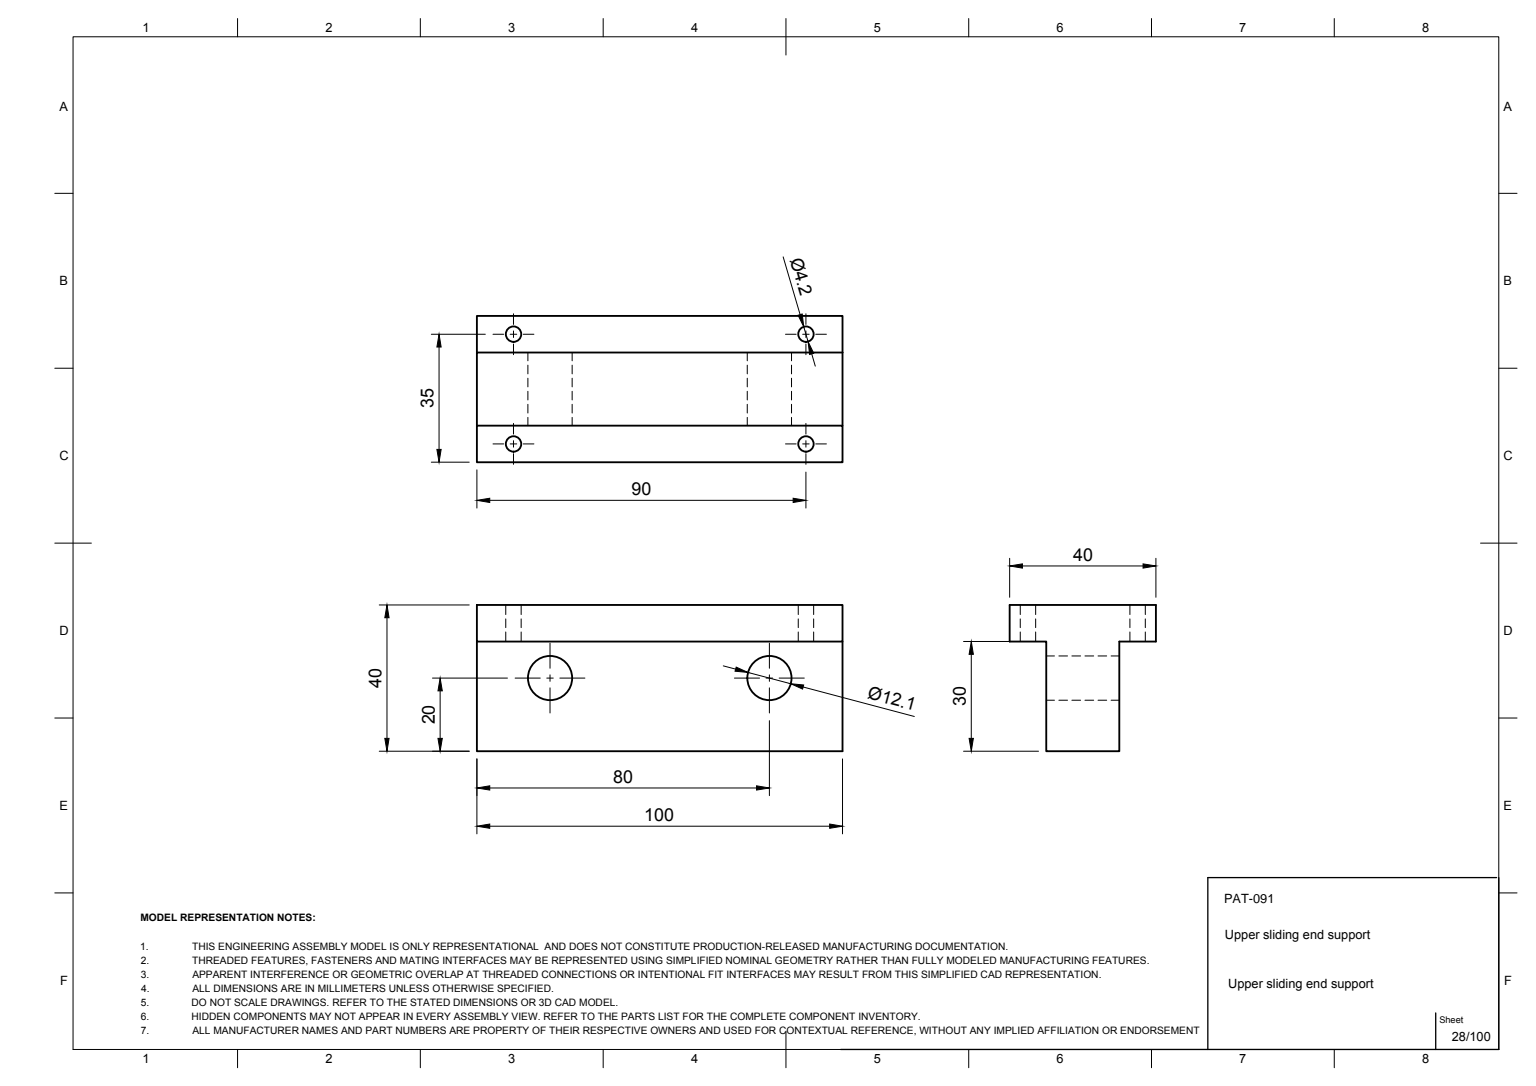
ISO-10303-21;
HEADER;
/* Generated by software containing ST-Developer
 * from STEP Tools, Inc. (www.steptools.com) 
 */

FILE_DESCRIPTION(
/* description */ ('PAT-091'),
/* implementation_level */ '2;1');

FILE_NAME(
/* name */ 'Upper sliding end support.step',
/* time_stamp */ '2026-10-27T15:34:44-07:00',
/* author */ (''),
/* organization */ (''),
/* preprocessor_version */ 'ST-DEVELOPER v20.2',
/* originating_system */ 'Autodesk Translation Framework v15.17.0.0',
/* authorisation */ '');

FILE_SCHEMA (('AUTOMOTIVE_DESIGN { 1 0 10303 214 3 1 1 }'));
ENDSEC;

DATA;
#10=MECHANICAL_DESIGN_GEOMETRIC_PRESENTATION_REPRESENTATION('',(#991),#25100);
#771=SHAPE_REPRESENTATION_RELATIONSHIP('SRR','None',#25533,#881);
#881=ADVANCED_BREP_SHAPE_REPRESENTATION('',(#1114),#25003);
#991=STYLED_ITEM('',(#26184),#1114);
#1114=MANIFOLD_SOLID_BREP('Body1',#13269);
#1365=FACE_BOUND('',#3226,.T.);
#1366=FACE_BOUND('',#3227,.T.);
#1367=FACE_BOUND('',#3231,.T.);
#1368=FACE_BOUND('',#3232,.T.);
#1369=FACE_BOUND('',#3234,.T.);
#1370=FACE_BOUND('',#3235,.T.);
#1371=FACE_BOUND('',#3241,.T.);
#1372=FACE_BOUND('',#3242,.T.);
#1373=FACE_BOUND('',#3244,.T.);
#1374=FACE_BOUND('',#3245,.T.);
#1375=FACE_BOUND('',#3246,.T.);
#1376=FACE_BOUND('',#3247,.T.);
#1736=PLANE('',#14996);
#1737=PLANE('',#14997);
#1738=PLANE('',#14998);
#1739=PLANE('',#14999);
#1740=PLANE('',#15000);
#1741=PLANE('',#15003);
#1742=PLANE('',#15008);
#1743=PLANE('',#15009);
#1744=PLANE('',#15010);
#1745=PLANE('',#15011);
#2253=FACE_OUTER_BOUND('',#3221,.T.);
#2254=FACE_OUTER_BOUND('',#3222,.T.);
#2255=FACE_OUTER_BOUND('',#3223,.T.);
#2256=FACE_OUTER_BOUND('',#3224,.T.);
#2257=FACE_OUTER_BOUND('',#3225,.T.);
#2258=FACE_OUTER_BOUND('',#3228,.T.);
#2259=FACE_OUTER_BOUND('',#3229,.T.);
#2260=FACE_OUTER_BOUND('',#3230,.T.);
#2261=FACE_OUTER_BOUND('',#3233,.T.);
#2262=FACE_OUTER_BOUND('',#3236,.T.);
#2263=FACE_OUTER_BOUND('',#3237,.T.);
#2264=FACE_OUTER_BOUND('',#3238,.T.);
#2265=FACE_OUTER_BOUND('',#3239,.T.);
#2266=FACE_OUTER_BOUND('',#3240,.T.);
#2267=FACE_OUTER_BOUND('',#3243,.T.);
#2268=FACE_OUTER_BOUND('',#3248,.T.);
#3221=EDGE_LOOP('',(#9806,#9807,#9808,#9809));
#3222=EDGE_LOOP('',(#9810,#9811,#9812,#9813));
#3223=EDGE_LOOP('',(#9814,#9815,#9816,#9817));
#3224=EDGE_LOOP('',(#9818,#9819,#9820,#9821));
#3225=EDGE_LOOP('',(#9822,#9823,#9824,#9825));
#3226=EDGE_LOOP('',(#9826));
#3227=EDGE_LOOP('',(#9827));
#3228=EDGE_LOOP('',(#9828,#9829,#9830,#9831));
#3229=EDGE_LOOP('',(#9832,#9833,#9834,#9835));
#3230=EDGE_LOOP('',(#9836,#9837,#9838,#9839));
#3231=EDGE_LOOP('',(#9840));
#3232=EDGE_LOOP('',(#9841));
#3233=EDGE_LOOP('',(#9842,#9843,#9844,#9845));
#3234=EDGE_LOOP('',(#9846));
#3235=EDGE_LOOP('',(#9847));
#3236=EDGE_LOOP('',(#9848,#9849,#9850,#9851,#9852,#9853,#9854,#9855));
#3237=EDGE_LOOP('',(#9856,#9857,#9858,#9859));
#3238=EDGE_LOOP('',(#9860,#9861,#9862,#9863));
#3239=EDGE_LOOP('',(#9864,#9865,#9866,#9867,#9868,#9869,#9870,#9871));
#3240=EDGE_LOOP('',(#9872,#9873,#9874,#9875));
#3241=EDGE_LOOP('',(#9876));
#3242=EDGE_LOOP('',(#9877));
#3243=EDGE_LOOP('',(#9878,#9879,#9880,#9881));
#3244=EDGE_LOOP('',(#9882));
#3245=EDGE_LOOP('',(#9883));
#3246=EDGE_LOOP('',(#9884));
#3247=EDGE_LOOP('',(#9885));
#3248=EDGE_LOOP('',(#9886,#9887,#9888,#9889));
#4356=LINE('',#21886,#5096);
#4357=LINE('',#21892,#5097);
#4358=LINE('',#21898,#5098);
#4359=LINE('',#21904,#5099);
#4360=LINE('',#21909,#5100);
#4361=LINE('',#21911,#5101);
#4362=LINE('',#21913,#5102);
#4363=LINE('',#21914,#5103);
#4364=LINE('',#21918,#5104);
#4365=LINE('',#21920,#5105);
#4366=LINE('',#21922,#5106);
#4367=LINE('',#21923,#5107);
#4368=LINE('',#21926,#5108);
#4369=LINE('',#21928,#5109);
#4370=LINE('',#21929,#5110);
#4371=LINE('',#21933,#5111);
#4372=LINE('',#21934,#5112);
#4373=LINE('',#21935,#5113);
#4374=LINE('',#21938,#5114);
#4375=LINE('',#21940,#5115);
#4376=LINE('',#21941,#5116);
#4377=LINE('',#21948,#5117);
#4378=LINE('',#21949,#5118);
#4379=LINE('',#21950,#5119);
#4380=LINE('',#21954,#5120);
#4381=LINE('',#21958,#5121);
#4382=LINE('',#21961,#5122);
#4383=LINE('',#21962,#5123);
#4384=LINE('',#21963,#5124);
#4385=LINE('',#21965,#5125);
#5096=VECTOR('',#17502,0.210000000000001);
#5097=VECTOR('',#17509,0.210000000000001);
#5098=VECTOR('',#17516,0.210000000000001);
#5099=VECTOR('',#17523,0.210000000000001);
#5100=VECTOR('',#17528,1.);
#5101=VECTOR('',#17529,1.);
#5102=VECTOR('',#17530,1.);
#5103=VECTOR('',#17531,1.);
#5104=VECTOR('',#17534,1.);
#5105=VECTOR('',#17535,1.);
#5106=VECTOR('',#17536,1.);
#5107=VECTOR('',#17537,1.);
#5108=VECTOR('',#17540,1.);
#5109=VECTOR('',#17541,1.);
#5110=VECTOR('',#17542,1.);
#5111=VECTOR('',#17545,1.);
#5112=VECTOR('',#17546,1.);
#5113=VECTOR('',#17547,1.);
#5114=VECTOR('',#17550,1.);
#5115=VECTOR('',#17551,1.);
#5116=VECTOR('',#17552,1.);
#5117=VECTOR('',#17559,1.);
#5118=VECTOR('',#17560,1.);
#5119=VECTOR('',#17561,1.);
#5120=VECTOR('',#17566,0.605);
#5121=VECTOR('',#17571,0.605);
#5122=VECTOR('',#17574,1.);
#5123=VECTOR('',#17575,1.);
#5124=VECTOR('',#17576,1.);
#5125=VECTOR('',#17579,1.);
#5789=CIRCLE('',#14985,0.210000000000001);
#5790=CIRCLE('',#14986,0.210000000000001);
#5791=CIRCLE('',#14988,0.210000000000001);
#5792=CIRCLE('',#14989,0.210000000000001);
#5793=CIRCLE('',#14991,0.210000000000001);
#5794=CIRCLE('',#14992,0.210000000000001);
#5795=CIRCLE('',#14994,0.210000000000001);
#5796=CIRCLE('',#14995,0.210000000000001);
#5797=CIRCLE('',#15001,0.605);
#5798=CIRCLE('',#15002,0.605);
#5799=CIRCLE('',#15005,0.605);
#5800=CIRCLE('',#15007,0.605);
#6660=VERTEX_POINT('',#21883);
#6661=VERTEX_POINT('',#21885);
#6662=VERTEX_POINT('',#21889);
#6663=VERTEX_POINT('',#21891);
#6664=VERTEX_POINT('',#21895);
#6665=VERTEX_POINT('',#21897);
#6666=VERTEX_POINT('',#21901);
#6667=VERTEX_POINT('',#21903);
#6668=VERTEX_POINT('',#21907);
#6669=VERTEX_POINT('',#21908);
#6670=VERTEX_POINT('',#21910);
#6671=VERTEX_POINT('',#21912);
#6672=VERTEX_POINT('',#21916);
#6673=VERTEX_POINT('',#21917);
#6674=VERTEX_POINT('',#21919);
#6675=VERTEX_POINT('',#21921);
#6676=VERTEX_POINT('',#21925);
#6677=VERTEX_POINT('',#21927);
#6678=VERTEX_POINT('',#21931);
#6679=VERTEX_POINT('',#21932);
#6680=VERTEX_POINT('',#21937);
#6681=VERTEX_POINT('',#21939);
#6682=VERTEX_POINT('',#21942);
#6683=VERTEX_POINT('',#21944);
#6684=VERTEX_POINT('',#21947);
#6685=VERTEX_POINT('',#21952);
#6686=VERTEX_POINT('',#21956);
#6687=VERTEX_POINT('',#21960);
#7838=EDGE_CURVE('',#6660,#6660,#5789,.T.);
#7839=EDGE_CURVE('',#6660,#6661,#4356,.T.);
#7840=EDGE_CURVE('',#6661,#6661,#5790,.T.);
#7841=EDGE_CURVE('',#6662,#6662,#5791,.T.);
#7842=EDGE_CURVE('',#6662,#6663,#4357,.T.);
#7843=EDGE_CURVE('',#6663,#6663,#5792,.T.);
#7844=EDGE_CURVE('',#6664,#6664,#5793,.T.);
#7845=EDGE_CURVE('',#6664,#6665,#4358,.T.);
#7846=EDGE_CURVE('',#6665,#6665,#5794,.T.);
#7847=EDGE_CURVE('',#6666,#6666,#5795,.T.);
#7848=EDGE_CURVE('',#6666,#6667,#4359,.T.);
#7849=EDGE_CURVE('',#6667,#6667,#5796,.T.);
#7850=EDGE_CURVE('',#6668,#6669,#4360,.T.);
#7851=EDGE_CURVE('',#6670,#6668,#4361,.T.);
#7852=EDGE_CURVE('',#6671,#6670,#4362,.T.);
#7853=EDGE_CURVE('',#6669,#6671,#4363,.T.);
#7854=EDGE_CURVE('',#6672,#6673,#4364,.T.);
#7855=EDGE_CURVE('',#6673,#6674,#4365,.T.);
#7856=EDGE_CURVE('',#6675,#6674,#4366,.T.);
#7857=EDGE_CURVE('',#6672,#6675,#4367,.T.);
#7858=EDGE_CURVE('',#6670,#6676,#4368,.T.);
#7859=EDGE_CURVE('',#6677,#6676,#4369,.T.);
#7860=EDGE_CURVE('',#6671,#6677,#4370,.T.);
#7861=EDGE_CURVE('',#6678,#6679,#4371,.T.);
#7862=EDGE_CURVE('',#6673,#6678,#4372,.T.);
#7863=EDGE_CURVE('',#6679,#6672,#4373,.T.);
#7864=EDGE_CURVE('',#6680,#6679,#4374,.T.);
#7865=EDGE_CURVE('',#6680,#6681,#4375,.T.);
#7866=EDGE_CURVE('',#6681,#6678,#4376,.T.);
#7867=EDGE_CURVE('',#6682,#6682,#5797,.T.);
#7868=EDGE_CURVE('',#6683,#6683,#5798,.T.);
#7869=EDGE_CURVE('',#6684,#6668,#4377,.T.);
#7870=EDGE_CURVE('',#6684,#6680,#4378,.T.);
#7871=EDGE_CURVE('',#6676,#6675,#4379,.T.);
#7872=EDGE_CURVE('',#6685,#6685,#5799,.T.);
#7873=EDGE_CURVE('',#6685,#6683,#4380,.T.);
#7874=EDGE_CURVE('',#6686,#6686,#5800,.T.);
#7875=EDGE_CURVE('',#6686,#6682,#4381,.T.);
#7876=EDGE_CURVE('',#6681,#6687,#4382,.T.);
#7877=EDGE_CURVE('',#6687,#6669,#4383,.T.);
#7878=EDGE_CURVE('',#6674,#6677,#4384,.T.);
#7879=EDGE_CURVE('',#6687,#6684,#4385,.T.);
#9806=ORIENTED_EDGE('',*,*,#7838,.F.);
#9807=ORIENTED_EDGE('',*,*,#7839,.T.);
#9808=ORIENTED_EDGE('',*,*,#7840,.F.);
#9809=ORIENTED_EDGE('',*,*,#7839,.F.);
#9810=ORIENTED_EDGE('',*,*,#7841,.F.);
#9811=ORIENTED_EDGE('',*,*,#7842,.T.);
#9812=ORIENTED_EDGE('',*,*,#7843,.F.);
#9813=ORIENTED_EDGE('',*,*,#7842,.F.);
#9814=ORIENTED_EDGE('',*,*,#7844,.F.);
#9815=ORIENTED_EDGE('',*,*,#7845,.T.);
#9816=ORIENTED_EDGE('',*,*,#7846,.F.);
#9817=ORIENTED_EDGE('',*,*,#7845,.F.);
#9818=ORIENTED_EDGE('',*,*,#7847,.F.);
#9819=ORIENTED_EDGE('',*,*,#7848,.T.);
#9820=ORIENTED_EDGE('',*,*,#7849,.F.);
#9821=ORIENTED_EDGE('',*,*,#7848,.F.);
#9822=ORIENTED_EDGE('',*,*,#7850,.F.);
#9823=ORIENTED_EDGE('',*,*,#7851,.F.);
#9824=ORIENTED_EDGE('',*,*,#7852,.F.);
#9825=ORIENTED_EDGE('',*,*,#7853,.F.);
#9826=ORIENTED_EDGE('',*,*,#7841,.T.);
#9827=ORIENTED_EDGE('',*,*,#7844,.T.);
#9828=ORIENTED_EDGE('',*,*,#7854,.T.);
#9829=ORIENTED_EDGE('',*,*,#7855,.T.);
#9830=ORIENTED_EDGE('',*,*,#7856,.F.);
#9831=ORIENTED_EDGE('',*,*,#7857,.F.);
#9832=ORIENTED_EDGE('',*,*,#7852,.T.);
#9833=ORIENTED_EDGE('',*,*,#7858,.T.);
#9834=ORIENTED_EDGE('',*,*,#7859,.F.);
#9835=ORIENTED_EDGE('',*,*,#7860,.F.);
#9836=ORIENTED_EDGE('',*,*,#7861,.F.);
#9837=ORIENTED_EDGE('',*,*,#7862,.F.);
#9838=ORIENTED_EDGE('',*,*,#7854,.F.);
#9839=ORIENTED_EDGE('',*,*,#7863,.F.);
#9840=ORIENTED_EDGE('',*,*,#7838,.T.);
#9841=ORIENTED_EDGE('',*,*,#7847,.T.);
#9842=ORIENTED_EDGE('',*,*,#7861,.T.);
#9843=ORIENTED_EDGE('',*,*,#7864,.F.);
#9844=ORIENTED_EDGE('',*,*,#7865,.T.);
#9845=ORIENTED_EDGE('',*,*,#7866,.T.);
#9846=ORIENTED_EDGE('',*,*,#7867,.T.);
#9847=ORIENTED_EDGE('',*,*,#7868,.T.);
#9848=ORIENTED_EDGE('',*,*,#7869,.F.);
#9849=ORIENTED_EDGE('',*,*,#7870,.T.);
#9850=ORIENTED_EDGE('',*,*,#7864,.T.);
#9851=ORIENTED_EDGE('',*,*,#7863,.T.);
#9852=ORIENTED_EDGE('',*,*,#7857,.T.);
#9853=ORIENTED_EDGE('',*,*,#7871,.F.);
#9854=ORIENTED_EDGE('',*,*,#7858,.F.);
#9855=ORIENTED_EDGE('',*,*,#7851,.T.);
#9856=ORIENTED_EDGE('',*,*,#7872,.F.);
#9857=ORIENTED_EDGE('',*,*,#7873,.T.);
#9858=ORIENTED_EDGE('',*,*,#7868,.F.);
#9859=ORIENTED_EDGE('',*,*,#7873,.F.);
#9860=ORIENTED_EDGE('',*,*,#7874,.F.);
#9861=ORIENTED_EDGE('',*,*,#7875,.T.);
#9862=ORIENTED_EDGE('',*,*,#7867,.F.);
#9863=ORIENTED_EDGE('',*,*,#7875,.F.);
#9864=ORIENTED_EDGE('',*,*,#7866,.F.);
#9865=ORIENTED_EDGE('',*,*,#7876,.T.);
#9866=ORIENTED_EDGE('',*,*,#7877,.T.);
#9867=ORIENTED_EDGE('',*,*,#7853,.T.);
#9868=ORIENTED_EDGE('',*,*,#7860,.T.);
#9869=ORIENTED_EDGE('',*,*,#7878,.F.);
#9870=ORIENTED_EDGE('',*,*,#7855,.F.);
#9871=ORIENTED_EDGE('',*,*,#7862,.T.);
#9872=ORIENTED_EDGE('',*,*,#7850,.T.);
#9873=ORIENTED_EDGE('',*,*,#7877,.F.);
#9874=ORIENTED_EDGE('',*,*,#7879,.T.);
#9875=ORIENTED_EDGE('',*,*,#7869,.T.);
#9876=ORIENTED_EDGE('',*,*,#7872,.T.);
#9877=ORIENTED_EDGE('',*,*,#7874,.T.);
#9878=ORIENTED_EDGE('',*,*,#7871,.T.);
#9879=ORIENTED_EDGE('',*,*,#7856,.T.);
#9880=ORIENTED_EDGE('',*,*,#7878,.T.);
#9881=ORIENTED_EDGE('',*,*,#7859,.T.);
#9882=ORIENTED_EDGE('',*,*,#7840,.T.);
#9883=ORIENTED_EDGE('',*,*,#7843,.T.);
#9884=ORIENTED_EDGE('',*,*,#7846,.T.);
#9885=ORIENTED_EDGE('',*,*,#7849,.T.);
#9886=ORIENTED_EDGE('',*,*,#7879,.F.);
#9887=ORIENTED_EDGE('',*,*,#7876,.F.);
#9888=ORIENTED_EDGE('',*,*,#7865,.F.);
#9889=ORIENTED_EDGE('',*,*,#7870,.F.);
#12165=CYLINDRICAL_SURFACE('',#14984,0.210000000000001);
#12166=CYLINDRICAL_SURFACE('',#14987,0.210000000000001);
#12167=CYLINDRICAL_SURFACE('',#14990,0.210000000000001);
#12168=CYLINDRICAL_SURFACE('',#14993,0.210000000000001);
#12169=CYLINDRICAL_SURFACE('',#15004,0.605);
#12170=CYLINDRICAL_SURFACE('',#15006,0.605);
#12620=ADVANCED_FACE('',(#2253),#12165,.F.);
#12621=ADVANCED_FACE('',(#2254),#12166,.F.);
#12622=ADVANCED_FACE('',(#2255),#12167,.F.);
#12623=ADVANCED_FACE('',(#2256),#12168,.F.);
#12624=ADVANCED_FACE('',(#2257,#1365,#1366),#1736,.F.);
#12625=ADVANCED_FACE('',(#2258),#1737,.T.);
#12626=ADVANCED_FACE('',(#2259),#1738,.T.);
#12627=ADVANCED_FACE('',(#2260,#1367,#1368),#1739,.F.);
#12628=ADVANCED_FACE('',(#2261,#1369,#1370),#1740,.T.);
#12629=ADVANCED_FACE('',(#2262),#1741,.T.);
#12630=ADVANCED_FACE('',(#2263),#12169,.F.);
#12631=ADVANCED_FACE('',(#2264),#12170,.F.);
#12632=ADVANCED_FACE('',(#2265),#1742,.T.);
#12633=ADVANCED_FACE('',(#2266,#1371,#1372),#1743,.T.);
#12634=ADVANCED_FACE('',(#2267,#1373,#1374,#1375,#1376),#1744,.T.);
#12635=ADVANCED_FACE('',(#2268),#1745,.F.);
#13269=CLOSED_SHELL('',(#12620,#12621,#12622,#12623,#12624,#12625,#12626,
#12627,#12628,#12629,#12630,#12631,#12632,#12633,#12634,#12635));
#14983=AXIS2_PLACEMENT_3D('',#21881,#17496,#17497);
#14984=AXIS2_PLACEMENT_3D('',#21882,#17498,#17499);
#14985=AXIS2_PLACEMENT_3D('',#21884,#17500,#17501);
#14986=AXIS2_PLACEMENT_3D('',#21887,#17503,#17504);
#14987=AXIS2_PLACEMENT_3D('',#21888,#17505,#17506);
#14988=AXIS2_PLACEMENT_3D('',#21890,#17507,#17508);
#14989=AXIS2_PLACEMENT_3D('',#21893,#17510,#17511);
#14990=AXIS2_PLACEMENT_3D('',#21894,#17512,#17513);
#14991=AXIS2_PLACEMENT_3D('',#21896,#17514,#17515);
#14992=AXIS2_PLACEMENT_3D('',#21899,#17517,#17518);
#14993=AXIS2_PLACEMENT_3D('',#21900,#17519,#17520);
#14994=AXIS2_PLACEMENT_3D('',#21902,#17521,#17522);
#14995=AXIS2_PLACEMENT_3D('',#21905,#17524,#17525);
#14996=AXIS2_PLACEMENT_3D('',#21906,#17526,#17527);
#14997=AXIS2_PLACEMENT_3D('',#21915,#17532,#17533);
#14998=AXIS2_PLACEMENT_3D('',#21924,#17538,#17539);
#14999=AXIS2_PLACEMENT_3D('',#21930,#17543,#17544);
#15000=AXIS2_PLACEMENT_3D('',#21936,#17548,#17549);
#15001=AXIS2_PLACEMENT_3D('',#21943,#17553,#17554);
#15002=AXIS2_PLACEMENT_3D('',#21945,#17555,#17556);
#15003=AXIS2_PLACEMENT_3D('',#21946,#17557,#17558);
#15004=AXIS2_PLACEMENT_3D('',#21951,#17562,#17563);
#15005=AXIS2_PLACEMENT_3D('',#21953,#17564,#17565);
#15006=AXIS2_PLACEMENT_3D('',#21955,#17567,#17568);
#15007=AXIS2_PLACEMENT_3D('',#21957,#17569,#17570);
#15008=AXIS2_PLACEMENT_3D('',#21959,#17572,#17573);
#15009=AXIS2_PLACEMENT_3D('',#21964,#17577,#17578);
#15010=AXIS2_PLACEMENT_3D('',#21966,#17580,#17581);
#15011=AXIS2_PLACEMENT_3D('',#21967,#17582,#17583);
#17496=DIRECTION('axis',(0.,0.,1.));
#17497=DIRECTION('refdir',(1.,0.,0.));
#17498=DIRECTION('center_axis',(0.,0.,1.));
#17499=DIRECTION('ref_axis',(1.,0.,0.));
#17500=DIRECTION('center_axis',(0.,0.,1.));
#17501=DIRECTION('ref_axis',(1.,0.,0.));
#17502=DIRECTION('',(0.,0.,1.));
#17503=DIRECTION('center_axis',(0.,0.,-1.));
#17504=DIRECTION('ref_axis',(1.,0.,0.));
#17505=DIRECTION('center_axis',(0.,0.,1.));
#17506=DIRECTION('ref_axis',(1.,0.,0.));
#17507=DIRECTION('center_axis',(0.,0.,1.));
#17508=DIRECTION('ref_axis',(1.,0.,0.));
#17509=DIRECTION('',(0.,0.,1.));
#17510=DIRECTION('center_axis',(0.,0.,-1.));
#17511=DIRECTION('ref_axis',(1.,0.,0.));
#17512=DIRECTION('center_axis',(0.,0.,1.));
#17513=DIRECTION('ref_axis',(1.,0.,0.));
#17514=DIRECTION('center_axis',(0.,0.,1.));
#17515=DIRECTION('ref_axis',(1.,0.,0.));
#17516=DIRECTION('',(0.,0.,1.));
#17517=DIRECTION('center_axis',(0.,0.,-1.));
#17518=DIRECTION('ref_axis',(1.,0.,0.));
#17519=DIRECTION('center_axis',(0.,0.,1.));
#17520=DIRECTION('ref_axis',(1.,0.,0.));
#17521=DIRECTION('center_axis',(0.,0.,1.));
#17522=DIRECTION('ref_axis',(1.,0.,0.));
#17523=DIRECTION('',(0.,0.,1.));
#17524=DIRECTION('center_axis',(0.,0.,-1.));
#17525=DIRECTION('ref_axis',(1.,0.,0.));
#17526=DIRECTION('center_axis',(0.,0.,1.));
#17527=DIRECTION('ref_axis',(1.,0.,0.));
#17528=DIRECTION('',(0.,1.,0.));
#17529=DIRECTION('',(1.,0.,0.));
#17530=DIRECTION('',(0.,-1.,0.));
#17531=DIRECTION('',(-1.,0.,0.));
#17532=DIRECTION('center_axis',(1.,0.,0.));
#17533=DIRECTION('ref_axis',(0.,1.,0.));
#17534=DIRECTION('',(0.,1.,0.));
#17535=DIRECTION('',(0.,0.,1.));
#17536=DIRECTION('',(0.,1.,0.));
#17537=DIRECTION('',(0.,0.,1.));
#17538=DIRECTION('center_axis',(-1.,0.,0.));
#17539=DIRECTION('ref_axis',(0.,-1.,0.));
#17540=DIRECTION('',(0.,0.,1.));
#17541=DIRECTION('',(0.,-1.,0.));
#17542=DIRECTION('',(0.,0.,1.));
#17543=DIRECTION('center_axis',(0.,0.,1.));
#17544=DIRECTION('ref_axis',(1.,0.,0.));
#17545=DIRECTION('',(0.,-1.,0.));
#17546=DIRECTION('',(-1.,0.,0.));
#17547=DIRECTION('',(1.,0.,0.));
#17548=DIRECTION('center_axis',(1.,0.,0.));
#17549=DIRECTION('ref_axis',(0.,1.,0.));
#17550=DIRECTION('',(0.,0.,1.));
#17551=DIRECTION('',(0.,1.,0.));
#17552=DIRECTION('',(0.,0.,1.));
#17553=DIRECTION('center_axis',(-1.,0.,0.));
#17554=DIRECTION('ref_axis',(0.,0.,-1.));
#17555=DIRECTION('center_axis',(-1.,0.,0.));
#17556=DIRECTION('ref_axis',(0.,0.,-1.));
#17557=DIRECTION('center_axis',(0.,-1.,0.));
#17558=DIRECTION('ref_axis',(1.,0.,0.));
#17559=DIRECTION('',(0.,0.,1.));
#17560=DIRECTION('',(1.,0.,0.));
#17561=DIRECTION('',(1.,0.,0.));
#17562=DIRECTION('center_axis',(1.,0.,0.));
#17563=DIRECTION('ref_axis',(0.,0.,-1.));
#17564=DIRECTION('center_axis',(1.,0.,0.));
#17565=DIRECTION('ref_axis',(0.,0.,-1.));
#17566=DIRECTION('',(1.,0.,0.));
#17567=DIRECTION('center_axis',(1.,0.,0.));
#17568=DIRECTION('ref_axis',(0.,0.,-1.));
#17569=DIRECTION('center_axis',(1.,0.,0.));
#17570=DIRECTION('ref_axis',(0.,0.,-1.));
#17571=DIRECTION('',(1.,0.,0.));
#17572=DIRECTION('center_axis',(0.,1.,0.));
#17573=DIRECTION('ref_axis',(-1.,0.,0.));
#17574=DIRECTION('',(-1.,0.,0.));
#17575=DIRECTION('',(0.,0.,1.));
#17576=DIRECTION('',(-1.,0.,0.));
#17577=DIRECTION('center_axis',(-1.,0.,0.));
#17578=DIRECTION('ref_axis',(0.,-1.,0.));
#17579=DIRECTION('',(0.,-1.,0.));
#17580=DIRECTION('center_axis',(0.,0.,1.));
#17581=DIRECTION('ref_axis',(1.,0.,0.));
#17582=DIRECTION('center_axis',(0.,0.,1.));
#17583=DIRECTION('ref_axis',(1.,0.,0.));
#21881=CARTESIAN_POINT('',(0.,0.,0.));
#21882=CARTESIAN_POINT('Origin',(46.5,-4.,16.9));
#21883=CARTESIAN_POINT('',(46.29,-4.,17.));
#21884=CARTESIAN_POINT('Origin',(46.5,-4.,17.));
#21885=CARTESIAN_POINT('',(46.29,-4.,18.));
#21886=CARTESIAN_POINT('',(46.29,-4.,16.9));
#21887=CARTESIAN_POINT('Origin',(46.5,-4.,18.));
#21888=CARTESIAN_POINT('Origin',(43.5,4.,16.9));
#21889=CARTESIAN_POINT('',(43.29,4.,17.));
#21890=CARTESIAN_POINT('Origin',(43.5,4.,17.));
#21891=CARTESIAN_POINT('',(43.29,4.,18.));
#21892=CARTESIAN_POINT('',(43.29,4.,16.9));
#21893=CARTESIAN_POINT('Origin',(43.5,4.,18.));
#21894=CARTESIAN_POINT('Origin',(43.5,-4.,16.9));
#21895=CARTESIAN_POINT('',(43.29,-4.,17.));
#21896=CARTESIAN_POINT('Origin',(43.5,-4.,17.));
#21897=CARTESIAN_POINT('',(43.29,-4.,18.));
#21898=CARTESIAN_POINT('',(43.29,-4.,16.9));
#21899=CARTESIAN_POINT('Origin',(43.5,-4.,18.));
#21900=CARTESIAN_POINT('Origin',(46.5,4.,16.9));
#21901=CARTESIAN_POINT('',(46.29,4.,17.));
#21902=CARTESIAN_POINT('Origin',(46.5,4.,17.));
#21903=CARTESIAN_POINT('',(46.29,4.,18.));
#21904=CARTESIAN_POINT('',(46.29,4.,16.9));
#21905=CARTESIAN_POINT('Origin',(46.5,4.,18.));
#21906=CARTESIAN_POINT('Origin',(45.,0.,17.));
#21907=CARTESIAN_POINT('',(44.,-5.,17.));
#21908=CARTESIAN_POINT('',(44.,5.,17.));
#21909=CARTESIAN_POINT('',(44.,2.5,17.));
#21910=CARTESIAN_POINT('',(43.,-5.,17.));
#21911=CARTESIAN_POINT('',(43.,-5.,17.));
#21912=CARTESIAN_POINT('',(43.,5.,17.));
#21913=CARTESIAN_POINT('',(43.,5.,17.));
#21914=CARTESIAN_POINT('',(47.,5.,17.));
#21915=CARTESIAN_POINT('Origin',(47.,-5.,17.));
#21916=CARTESIAN_POINT('',(47.,-5.,17.));
#21917=CARTESIAN_POINT('',(47.,5.,17.));
#21918=CARTESIAN_POINT('',(47.,-5.,17.));
#21919=CARTESIAN_POINT('',(47.,5.,18.));
#21920=CARTESIAN_POINT('',(47.,5.,17.));
#21921=CARTESIAN_POINT('',(47.,-5.,18.));
#21922=CARTESIAN_POINT('',(47.,-5.,18.));
#21923=CARTESIAN_POINT('',(47.,-5.,17.));
#21924=CARTESIAN_POINT('Origin',(43.,5.,17.));
#21925=CARTESIAN_POINT('',(43.,-5.,18.));
#21926=CARTESIAN_POINT('',(43.,-5.,17.));
#21927=CARTESIAN_POINT('',(43.,5.,18.));
#21928=CARTESIAN_POINT('',(43.,5.,18.));
#21929=CARTESIAN_POINT('',(43.,5.,17.));
#21930=CARTESIAN_POINT('Origin',(45.,0.,17.));
#21931=CARTESIAN_POINT('',(46.,5.,17.));
#21932=CARTESIAN_POINT('',(46.,-5.,17.));
#21933=CARTESIAN_POINT('',(46.,-2.5,17.));
#21934=CARTESIAN_POINT('',(47.,5.,17.));
#21935=CARTESIAN_POINT('',(43.,-5.,17.));
#21936=CARTESIAN_POINT('Origin',(46.,-5.,14.));
#21937=CARTESIAN_POINT('',(46.,-5.,14.));
#21938=CARTESIAN_POINT('',(46.,-5.,14.));
#21939=CARTESIAN_POINT('',(46.,5.,14.));
#21940=CARTESIAN_POINT('',(46.,-5.,14.));
#21941=CARTESIAN_POINT('',(46.,5.,14.));
#21942=CARTESIAN_POINT('',(46.,3.,16.605));
#21943=CARTESIAN_POINT('Origin',(46.,3.,16.));
#21944=CARTESIAN_POINT('',(46.,-3.,16.605));
#21945=CARTESIAN_POINT('Origin',(46.,-3.,16.));
#21946=CARTESIAN_POINT('Origin',(44.,-5.,14.));
#21947=CARTESIAN_POINT('',(44.,-5.,14.));
#21948=CARTESIAN_POINT('',(44.,-5.,14.));
#21949=CARTESIAN_POINT('',(44.,-5.,14.));
#21950=CARTESIAN_POINT('',(43.,-5.,18.));
#21951=CARTESIAN_POINT('Origin',(43.9,-3.,16.));
#21952=CARTESIAN_POINT('',(44.,-3.,16.605));
#21953=CARTESIAN_POINT('Origin',(44.,-3.,16.));
#21954=CARTESIAN_POINT('',(43.9,-3.,16.605));
#21955=CARTESIAN_POINT('Origin',(43.9,3.,16.));
#21956=CARTESIAN_POINT('',(44.,3.,16.605));
#21957=CARTESIAN_POINT('Origin',(44.,3.,16.));
#21958=CARTESIAN_POINT('',(43.9,3.,16.605));
#21959=CARTESIAN_POINT('Origin',(46.,5.,14.));
#21960=CARTESIAN_POINT('',(44.,5.,14.));
#21961=CARTESIAN_POINT('',(46.,5.,14.));
#21962=CARTESIAN_POINT('',(44.,5.,14.));
#21963=CARTESIAN_POINT('',(47.,5.,18.));
#21964=CARTESIAN_POINT('Origin',(44.,5.,14.));
#21965=CARTESIAN_POINT('',(44.,5.,14.));
#21966=CARTESIAN_POINT('Origin',(45.,0.,18.));
#21967=CARTESIAN_POINT('Origin',(45.,0.,14.));
#24882=UNCERTAINTY_MEASURE_WITH_UNIT(LENGTH_MEASURE(0.001),#25101,
'DISTANCE_ACCURACY_VALUE',
'Maximum model space distance between geometric entities at asserted c
onnectivities');
#24979=UNCERTAINTY_MEASURE_WITH_UNIT(LENGTH_MEASURE(0.001),#25101,
'DISTANCE_ACCURACY_VALUE',
'Maximum model space distance between geometric entities at asserted c
onnectivities');
#25003=(
GEOMETRIC_REPRESENTATION_CONTEXT(3)
GLOBAL_UNCERTAINTY_ASSIGNED_CONTEXT((#24882))
GLOBAL_UNIT_ASSIGNED_CONTEXT((#25101,#25103,#25104))
REPRESENTATION_CONTEXT('','3D')
);
#25100=(
GEOMETRIC_REPRESENTATION_CONTEXT(3)
GLOBAL_UNCERTAINTY_ASSIGNED_CONTEXT((#24979))
GLOBAL_UNIT_ASSIGNED_CONTEXT((#25101,#25103,#25104))
REPRESENTATION_CONTEXT('','3D')
);
#25101=(
LENGTH_UNIT()
NAMED_UNIT(*)
SI_UNIT(.CENTI.,.METRE.)
);
#25103=(
NAMED_UNIT(*)
PLANE_ANGLE_UNIT()
SI_UNIT($,.RADIAN.)
);
#25104=(
NAMED_UNIT(*)
SI_UNIT($,.STERADIAN.)
SOLID_ANGLE_UNIT()
);
#25128=SHAPE_DEFINITION_REPRESENTATION(#25248,#25533);
#25248=PRODUCT_DEFINITION_SHAPE('',$,#25654);
#25533=SHAPE_REPRESENTATION('',(#14983),#25003);
#25630=PRODUCT_DEFINITION_CONTEXT('part definition',#25992,'design');
#25654=PRODUCT_DEFINITION('Upper sliding end support',
'Upper sliding end support',#25774,#25630);
#25774=PRODUCT_DEFINITION_FORMATION('',$,#26017);
#25992=APPLICATION_CONTEXT(
'Core Data for Automotive Mechanical Design Process');
#25993=PRODUCT_CONTEXT('part definition',#25992,'mechanical');
#26017=PRODUCT('Upper sliding end support','Upper sliding end support',
'Upper sliding end support',(#25993));
#26178=COLOUR_RGB('Sky Blue',0.24,0.69,0.87);
#26179=FILL_AREA_STYLE_COLOUR('',#26178);
#26180=FILL_AREA_STYLE('',(#26179));
#26181=SURFACE_STYLE_FILL_AREA(#26180);
#26182=SURFACE_SIDE_STYLE('',(#26181));
#26183=SURFACE_STYLE_USAGE(.BOTH.,#26182);
#26184=PRESENTATION_STYLE_ASSIGNMENT((#26183));
ENDSEC;
END-ISO-10303-21;
